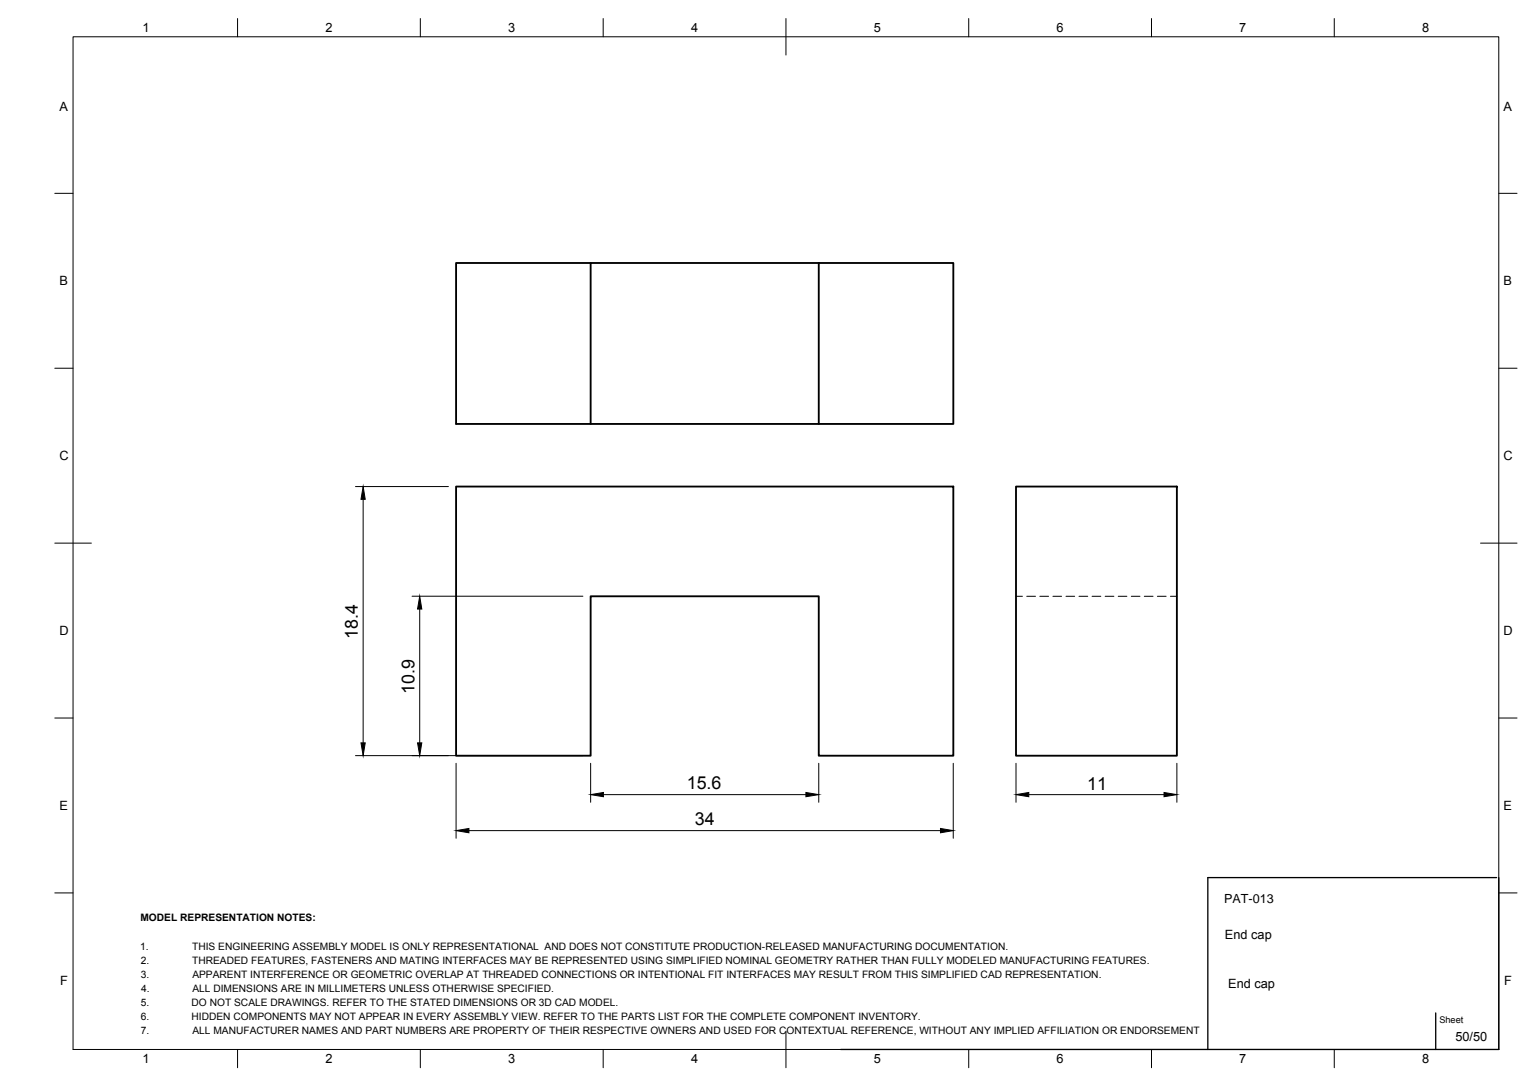
ISO-10303-21;
HEADER;
/* Generated by software containing ST-Developer
 * from STEP Tools, Inc. (www.steptools.com) 
 */

FILE_DESCRIPTION(
/* description */ ('Belt-driven linear axis on 2020 extrusion'),
/* implementation_level */ '2;1');

FILE_NAME(
/* name */ 'End cap.step',
/* time_stamp */ '2026-10-28T03:26:09-07:00',
/* author */ (''),
/* organization */ (''),
/* preprocessor_version */ 'ST-DEVELOPER v20.2',
/* originating_system */ 'Autodesk Translation Framework v15.17.0.0',
/* authorisation */ '');

FILE_SCHEMA (('AUTOMOTIVE_DESIGN { 1 0 10303 214 3 1 1 }'));
ENDSEC;

DATA;
#10=MECHANICAL_DESIGN_GEOMETRIC_PRESENTATION_REPRESENTATION('',(#661),#20096);
#559=SHAPE_REPRESENTATION_RELATIONSHIP('SRR','None',#20360,#605);
#605=ADVANCED_BREP_SHAPE_REPRESENTATION('',(#716),#20091);
#661=STYLED_ITEM('',(#20664),#716);
#716=MANIFOLD_SOLID_BREP('Body1',#10975);
#1205=PLANE('',#12588);
#1206=PLANE('',#12589);
#1207=PLANE('',#12590);
#1208=PLANE('',#12591);
#1209=PLANE('',#12592);
#1210=PLANE('',#12593);
#1211=PLANE('',#12594);
#1212=PLANE('',#12595);
#1213=PLANE('',#12596);
#1214=PLANE('',#12597);
#1807=FACE_OUTER_BOUND('',#2595,.T.);
#1808=FACE_OUTER_BOUND('',#2596,.T.);
#1809=FACE_OUTER_BOUND('',#2597,.T.);
#1810=FACE_OUTER_BOUND('',#2598,.T.);
#1811=FACE_OUTER_BOUND('',#2599,.T.);
#1812=FACE_OUTER_BOUND('',#2600,.T.);
#1813=FACE_OUTER_BOUND('',#2601,.T.);
#1814=FACE_OUTER_BOUND('',#2602,.T.);
#1815=FACE_OUTER_BOUND('',#2603,.T.);
#1816=FACE_OUTER_BOUND('',#2604,.T.);
#2595=EDGE_LOOP('',(#9825,#9826,#9827,#9828));
#2596=EDGE_LOOP('',(#9829,#9830,#9831,#9832));
#2597=EDGE_LOOP('',(#9833,#9834,#9835,#9836));
#2598=EDGE_LOOP('',(#9837,#9838,#9839,#9840));
#2599=EDGE_LOOP('',(#9841,#9842,#9843,#9844));
#2600=EDGE_LOOP('',(#9845,#9846,#9847,#9848));
#2601=EDGE_LOOP('',(#9849,#9850,#9851,#9852));
#2602=EDGE_LOOP('',(#9853,#9854,#9855,#9856));
#2603=EDGE_LOOP('',(#9857,#9858,#9859,#9860,#9861,#9862,#9863,#9864));
#2604=EDGE_LOOP('',(#9865,#9866,#9867,#9868,#9869,#9870,#9871,#9872));
#3424=LINE('',#19617,#4281);
#3425=LINE('',#19619,#4282);
#3426=LINE('',#19621,#4283);
#3427=LINE('',#19622,#4284);
#3428=LINE('',#19625,#4285);
#3429=LINE('',#19627,#4286);
#3430=LINE('',#19628,#4287);
#3431=LINE('',#19631,#4288);
#3432=LINE('',#19633,#4289);
#3433=LINE('',#19634,#4290);
#3434=LINE('',#19637,#4291);
#3435=LINE('',#19639,#4292);
#3436=LINE('',#19640,#4293);
#3437=LINE('',#19643,#4294);
#3438=LINE('',#19645,#4295);
#3439=LINE('',#19646,#4296);
#3440=LINE('',#19649,#4297);
#3441=LINE('',#19651,#4298);
#3442=LINE('',#19652,#4299);
#3443=LINE('',#19655,#4300);
#3444=LINE('',#19657,#4301);
#3445=LINE('',#19658,#4302);
#3446=LINE('',#19660,#4303);
#3447=LINE('',#19661,#4304);
#4281=VECTOR('',#15742,1.);
#4282=VECTOR('',#15743,1.);
#4283=VECTOR('',#15744,1.);
#4284=VECTOR('',#15745,1.);
#4285=VECTOR('',#15748,1.);
#4286=VECTOR('',#15749,1.);
#4287=VECTOR('',#15750,1.);
#4288=VECTOR('',#15753,1.);
#4289=VECTOR('',#15754,1.);
#4290=VECTOR('',#15755,1.);
#4291=VECTOR('',#15758,1.);
#4292=VECTOR('',#15759,1.);
#4293=VECTOR('',#15760,1.);
#4294=VECTOR('',#15763,1.);
#4295=VECTOR('',#15764,1.);
#4296=VECTOR('',#15765,1.);
#4297=VECTOR('',#15768,1.);
#4298=VECTOR('',#15769,1.);
#4299=VECTOR('',#15770,1.);
#4300=VECTOR('',#15773,1.);
#4301=VECTOR('',#15774,1.);
#4302=VECTOR('',#15775,1.);
#4303=VECTOR('',#15778,1.);
#4304=VECTOR('',#15779,1.);
#5761=VERTEX_POINT('',#19615);
#5762=VERTEX_POINT('',#19616);
#5763=VERTEX_POINT('',#19618);
#5764=VERTEX_POINT('',#19620);
#5765=VERTEX_POINT('',#19624);
#5766=VERTEX_POINT('',#19626);
#5767=VERTEX_POINT('',#19630);
#5768=VERTEX_POINT('',#19632);
#5769=VERTEX_POINT('',#19636);
#5770=VERTEX_POINT('',#19638);
#5771=VERTEX_POINT('',#19642);
#5772=VERTEX_POINT('',#19644);
#5773=VERTEX_POINT('',#19648);
#5774=VERTEX_POINT('',#19650);
#5775=VERTEX_POINT('',#19654);
#5776=VERTEX_POINT('',#19656);
#7127=EDGE_CURVE('',#5761,#5762,#3424,.T.);
#7128=EDGE_CURVE('',#5761,#5763,#3425,.T.);
#7129=EDGE_CURVE('',#5764,#5763,#3426,.T.);
#7130=EDGE_CURVE('',#5762,#5764,#3427,.T.);
#7131=EDGE_CURVE('',#5762,#5765,#3428,.T.);
#7132=EDGE_CURVE('',#5766,#5764,#3429,.T.);
#7133=EDGE_CURVE('',#5765,#5766,#3430,.T.);
#7134=EDGE_CURVE('',#5765,#5767,#3431,.T.);
#7135=EDGE_CURVE('',#5768,#5766,#3432,.T.);
#7136=EDGE_CURVE('',#5767,#5768,#3433,.T.);
#7137=EDGE_CURVE('',#5767,#5769,#3434,.T.);
#7138=EDGE_CURVE('',#5770,#5768,#3435,.T.);
#7139=EDGE_CURVE('',#5769,#5770,#3436,.T.);
#7140=EDGE_CURVE('',#5769,#5771,#3437,.T.);
#7141=EDGE_CURVE('',#5772,#5770,#3438,.T.);
#7142=EDGE_CURVE('',#5771,#5772,#3439,.T.);
#7143=EDGE_CURVE('',#5771,#5773,#3440,.T.);
#7144=EDGE_CURVE('',#5774,#5772,#3441,.T.);
#7145=EDGE_CURVE('',#5773,#5774,#3442,.T.);
#7146=EDGE_CURVE('',#5773,#5775,#3443,.T.);
#7147=EDGE_CURVE('',#5776,#5774,#3444,.T.);
#7148=EDGE_CURVE('',#5775,#5776,#3445,.T.);
#7149=EDGE_CURVE('',#5775,#5761,#3446,.T.);
#7150=EDGE_CURVE('',#5763,#5776,#3447,.T.);
#9825=ORIENTED_EDGE('',*,*,#7127,.F.);
#9826=ORIENTED_EDGE('',*,*,#7128,.T.);
#9827=ORIENTED_EDGE('',*,*,#7129,.F.);
#9828=ORIENTED_EDGE('',*,*,#7130,.F.);
#9829=ORIENTED_EDGE('',*,*,#7131,.F.);
#9830=ORIENTED_EDGE('',*,*,#7130,.T.);
#9831=ORIENTED_EDGE('',*,*,#7132,.F.);
#9832=ORIENTED_EDGE('',*,*,#7133,.F.);
#9833=ORIENTED_EDGE('',*,*,#7134,.F.);
#9834=ORIENTED_EDGE('',*,*,#7133,.T.);
#9835=ORIENTED_EDGE('',*,*,#7135,.F.);
#9836=ORIENTED_EDGE('',*,*,#7136,.F.);
#9837=ORIENTED_EDGE('',*,*,#7137,.F.);
#9838=ORIENTED_EDGE('',*,*,#7136,.T.);
#9839=ORIENTED_EDGE('',*,*,#7138,.F.);
#9840=ORIENTED_EDGE('',*,*,#7139,.F.);
#9841=ORIENTED_EDGE('',*,*,#7140,.F.);
#9842=ORIENTED_EDGE('',*,*,#7139,.T.);
#9843=ORIENTED_EDGE('',*,*,#7141,.F.);
#9844=ORIENTED_EDGE('',*,*,#7142,.F.);
#9845=ORIENTED_EDGE('',*,*,#7143,.F.);
#9846=ORIENTED_EDGE('',*,*,#7142,.T.);
#9847=ORIENTED_EDGE('',*,*,#7144,.F.);
#9848=ORIENTED_EDGE('',*,*,#7145,.F.);
#9849=ORIENTED_EDGE('',*,*,#7146,.F.);
#9850=ORIENTED_EDGE('',*,*,#7145,.T.);
#9851=ORIENTED_EDGE('',*,*,#7147,.F.);
#9852=ORIENTED_EDGE('',*,*,#7148,.F.);
#9853=ORIENTED_EDGE('',*,*,#7149,.F.);
#9854=ORIENTED_EDGE('',*,*,#7148,.T.);
#9855=ORIENTED_EDGE('',*,*,#7150,.F.);
#9856=ORIENTED_EDGE('',*,*,#7128,.F.);
#9857=ORIENTED_EDGE('',*,*,#7149,.T.);
#9858=ORIENTED_EDGE('',*,*,#7127,.T.);
#9859=ORIENTED_EDGE('',*,*,#7131,.T.);
#9860=ORIENTED_EDGE('',*,*,#7134,.T.);
#9861=ORIENTED_EDGE('',*,*,#7137,.T.);
#9862=ORIENTED_EDGE('',*,*,#7140,.T.);
#9863=ORIENTED_EDGE('',*,*,#7143,.T.);
#9864=ORIENTED_EDGE('',*,*,#7146,.T.);
#9865=ORIENTED_EDGE('',*,*,#7150,.T.);
#9866=ORIENTED_EDGE('',*,*,#7147,.T.);
#9867=ORIENTED_EDGE('',*,*,#7144,.T.);
#9868=ORIENTED_EDGE('',*,*,#7141,.T.);
#9869=ORIENTED_EDGE('',*,*,#7138,.T.);
#9870=ORIENTED_EDGE('',*,*,#7135,.T.);
#9871=ORIENTED_EDGE('',*,*,#7132,.T.);
#9872=ORIENTED_EDGE('',*,*,#7129,.T.);
#10858=ADVANCED_FACE('',(#1807),#1205,.T.);
#10859=ADVANCED_FACE('',(#1808),#1206,.T.);
#10860=ADVANCED_FACE('',(#1809),#1207,.T.);
#10861=ADVANCED_FACE('',(#1810),#1208,.T.);
#10862=ADVANCED_FACE('',(#1811),#1209,.T.);
#10863=ADVANCED_FACE('',(#1812),#1210,.T.);
#10864=ADVANCED_FACE('',(#1813),#1211,.T.);
#10865=ADVANCED_FACE('',(#1814),#1212,.T.);
#10866=ADVANCED_FACE('',(#1815),#1213,.T.);
#10867=ADVANCED_FACE('',(#1816),#1214,.T.);
#10975=CLOSED_SHELL('',(#10858,#10859,#10860,#10861,#10862,#10863,#10864,
#10865,#10866,#10867));
#12587=AXIS2_PLACEMENT_3D('',#19613,#15738,#15739);
#12588=AXIS2_PLACEMENT_3D('',#19614,#15740,#15741);
#12589=AXIS2_PLACEMENT_3D('',#19623,#15746,#15747);
#12590=AXIS2_PLACEMENT_3D('',#19629,#15751,#15752);
#12591=AXIS2_PLACEMENT_3D('',#19635,#15756,#15757);
#12592=AXIS2_PLACEMENT_3D('',#19641,#15761,#15762);
#12593=AXIS2_PLACEMENT_3D('',#19647,#15766,#15767);
#12594=AXIS2_PLACEMENT_3D('',#19653,#15771,#15772);
#12595=AXIS2_PLACEMENT_3D('',#19659,#15776,#15777);
#12596=AXIS2_PLACEMENT_3D('',#19662,#15780,#15781);
#12597=AXIS2_PLACEMENT_3D('',#19663,#15782,#15783);
#15738=DIRECTION('axis',(0.,0.,1.));
#15739=DIRECTION('refdir',(1.,0.,0.));
#15740=DIRECTION('center_axis',(0.,0.,-1.));
#15741=DIRECTION('ref_axis',(0.,-1.,0.));
#15742=DIRECTION('',(0.,1.,0.));
#15743=DIRECTION('',(-1.,0.,0.));
#15744=DIRECTION('',(0.,-1.,0.));
#15745=DIRECTION('',(-1.,0.,0.));
#15746=DIRECTION('center_axis',(0.,1.,0.));
#15747=DIRECTION('ref_axis',(0.,0.,-1.));
#15748=DIRECTION('',(0.,0.,1.));
#15749=DIRECTION('',(0.,0.,-1.));
#15750=DIRECTION('',(-1.,0.,0.));
#15751=DIRECTION('center_axis',(0.,0.,-1.));
#15752=DIRECTION('ref_axis',(0.,-1.,0.));
#15753=DIRECTION('',(0.,1.,0.));
#15754=DIRECTION('',(0.,-1.,0.));
#15755=DIRECTION('',(-1.,0.,0.));
#15756=DIRECTION('center_axis',(0.,-1.,0.));
#15757=DIRECTION('ref_axis',(0.,0.,1.));
#15758=DIRECTION('',(0.,0.,-1.));
#15759=DIRECTION('',(0.,0.,1.));
#15760=DIRECTION('',(-1.,0.,0.));
#15761=DIRECTION('center_axis',(0.,0.,-1.));
#15762=DIRECTION('ref_axis',(0.,-1.,0.));
#15763=DIRECTION('',(0.,1.,0.));
#15764=DIRECTION('',(0.,-1.,0.));
#15765=DIRECTION('',(-1.,0.,0.));
#15766=DIRECTION('center_axis',(0.,1.,0.));
#15767=DIRECTION('ref_axis',(0.,0.,-1.));
#15768=DIRECTION('',(0.,0.,1.));
#15769=DIRECTION('',(0.,0.,-1.));
#15770=DIRECTION('',(-1.,0.,0.));
#15771=DIRECTION('center_axis',(0.,0.,1.));
#15772=DIRECTION('ref_axis',(0.,1.,0.));
#15773=DIRECTION('',(0.,-1.,0.));
#15774=DIRECTION('',(0.,1.,0.));
#15775=DIRECTION('',(-1.,0.,0.));
#15776=DIRECTION('center_axis',(0.,-1.,0.));
#15777=DIRECTION('ref_axis',(0.,0.,1.));
#15778=DIRECTION('',(0.,0.,-1.));
#15779=DIRECTION('',(0.,0.,1.));
#15780=DIRECTION('center_axis',(1.,0.,0.));
#15781=DIRECTION('ref_axis',(0.,0.,-1.));
#15782=DIRECTION('center_axis',(-1.,0.,0.));
#15783=DIRECTION('ref_axis',(0.,0.,1.));
#19613=CARTESIAN_POINT('',(0.,0.,0.));
#19614=CARTESIAN_POINT('Origin',(-1.97,-0.78,0.46));
#19615=CARTESIAN_POINT('',(-1.97,-1.7,0.46));
#19616=CARTESIAN_POINT('',(-1.97,-0.78,0.46));
#19617=CARTESIAN_POINT('',(-1.97,-1.7,0.46));
#19618=CARTESIAN_POINT('',(-3.07,-1.7,0.46));
#19619=CARTESIAN_POINT('',(-1.97,-1.7,0.46));
#19620=CARTESIAN_POINT('',(-3.07,-0.78,0.46));
#19621=CARTESIAN_POINT('',(-3.07,-1.7,0.46));
#19622=CARTESIAN_POINT('',(-1.97,-0.78,0.46));
#19623=CARTESIAN_POINT('Origin',(-1.97,-0.78,1.55));
#19624=CARTESIAN_POINT('',(-1.97,-0.78,1.55));
#19625=CARTESIAN_POINT('',(-1.97,-0.78,0.46));
#19626=CARTESIAN_POINT('',(-3.07,-0.78,1.55));
#19627=CARTESIAN_POINT('',(-3.07,-0.78,0.46));
#19628=CARTESIAN_POINT('',(-1.97,-0.78,1.55));
#19629=CARTESIAN_POINT('Origin',(-1.97,0.78,1.55));
#19630=CARTESIAN_POINT('',(-1.97,0.78,1.55));
#19631=CARTESIAN_POINT('',(-1.97,-0.78,1.55));
#19632=CARTESIAN_POINT('',(-3.07,0.78,1.55));
#19633=CARTESIAN_POINT('',(-3.07,-0.78,1.55));
#19634=CARTESIAN_POINT('',(-1.97,0.78,1.55));
#19635=CARTESIAN_POINT('Origin',(-1.97,0.78,0.46));
#19636=CARTESIAN_POINT('',(-1.97,0.78,0.46));
#19637=CARTESIAN_POINT('',(-1.97,0.78,1.55));
#19638=CARTESIAN_POINT('',(-3.07,0.78,0.46));
#19639=CARTESIAN_POINT('',(-3.07,0.78,1.55));
#19640=CARTESIAN_POINT('',(-1.97,0.78,0.46));
#19641=CARTESIAN_POINT('Origin',(-1.97,1.7,0.46));
#19642=CARTESIAN_POINT('',(-1.97,1.7,0.46));
#19643=CARTESIAN_POINT('',(-1.97,0.78,0.46));
#19644=CARTESIAN_POINT('',(-3.07,1.7,0.46));
#19645=CARTESIAN_POINT('',(-3.07,0.78,0.46));
#19646=CARTESIAN_POINT('',(-1.97,1.7,0.46));
#19647=CARTESIAN_POINT('Origin',(-1.97,1.7,2.3));
#19648=CARTESIAN_POINT('',(-1.97,1.7,2.3));
#19649=CARTESIAN_POINT('',(-1.97,1.7,0.46));
#19650=CARTESIAN_POINT('',(-3.07,1.7,2.3));
#19651=CARTESIAN_POINT('',(-3.07,1.7,0.46));
#19652=CARTESIAN_POINT('',(-1.97,1.7,2.3));
#19653=CARTESIAN_POINT('Origin',(-1.97,-1.7,2.3));
#19654=CARTESIAN_POINT('',(-1.97,-1.7,2.3));
#19655=CARTESIAN_POINT('',(-1.97,1.7,2.3));
#19656=CARTESIAN_POINT('',(-3.07,-1.7,2.3));
#19657=CARTESIAN_POINT('',(-3.07,1.7,2.3));
#19658=CARTESIAN_POINT('',(-1.97,-1.7,2.3));
#19659=CARTESIAN_POINT('Origin',(-1.97,-1.7,0.46));
#19660=CARTESIAN_POINT('',(-1.97,-1.7,2.3));
#19661=CARTESIAN_POINT('',(-3.07,-1.7,2.3));
#19662=CARTESIAN_POINT('Origin',(-1.97,0.,1.38));
#19663=CARTESIAN_POINT('Origin',(-3.07,0.,1.38));
#20037=UNCERTAINTY_MEASURE_WITH_UNIT(LENGTH_MEASURE(0.001),#20097,
'DISTANCE_ACCURACY_VALUE',
'Maximum model space distance between geometric entities at asserted c
onnectivities');
#20042=UNCERTAINTY_MEASURE_WITH_UNIT(LENGTH_MEASURE(0.001),#20097,
'DISTANCE_ACCURACY_VALUE',
'Maximum model space distance between geometric entities at asserted c
onnectivities');
#20091=(
GEOMETRIC_REPRESENTATION_CONTEXT(3)
GLOBAL_UNCERTAINTY_ASSIGNED_CONTEXT((#20037))
GLOBAL_UNIT_ASSIGNED_CONTEXT((#20097,#20099,#20100))
REPRESENTATION_CONTEXT('','3D')
);
#20096=(
GEOMETRIC_REPRESENTATION_CONTEXT(3)
GLOBAL_UNCERTAINTY_ASSIGNED_CONTEXT((#20042))
GLOBAL_UNIT_ASSIGNED_CONTEXT((#20097,#20099,#20100))
REPRESENTATION_CONTEXT('','3D')
);
#20097=(
LENGTH_UNIT()
NAMED_UNIT(*)
SI_UNIT(.CENTI.,.METRE.)
);
#20099=(
NAMED_UNIT(*)
PLANE_ANGLE_UNIT()
SI_UNIT($,.RADIAN.)
);
#20100=(
NAMED_UNIT(*)
SI_UNIT($,.STERADIAN.)
SOLID_ANGLE_UNIT()
);
#20149=SHAPE_DEFINITION_REPRESENTATION(#20207,#20360);
#20207=PRODUCT_DEFINITION_SHAPE('',$,#20414);
#20360=SHAPE_REPRESENTATION('',(#12587),#20091);
#20365=PRODUCT_DEFINITION_CONTEXT('part definition',#20526,'design');
#20414=PRODUCT_DEFINITION('End cap','End cap',#20467,#20365);
#20467=PRODUCT_DEFINITION_FORMATION('',$,#20576);
#20526=APPLICATION_CONTEXT(
'Core Data for Automotive Mechanical Design Process');
#20527=PRODUCT_CONTEXT('part definition',#20526,'mechanical');
#20576=PRODUCT('End cap','End cap','End cap',(#20527));
#20658=COLOUR_RGB('Off White',0.89,0.88,0.83);
#20659=FILL_AREA_STYLE_COLOUR('',#20658);
#20660=FILL_AREA_STYLE('',(#20659));
#20661=SURFACE_STYLE_FILL_AREA(#20660);
#20662=SURFACE_SIDE_STYLE('',(#20661));
#20663=SURFACE_STYLE_USAGE(.BOTH.,#20662);
#20664=PRESENTATION_STYLE_ASSIGNMENT((#20663));
ENDSEC;
END-ISO-10303-21;
